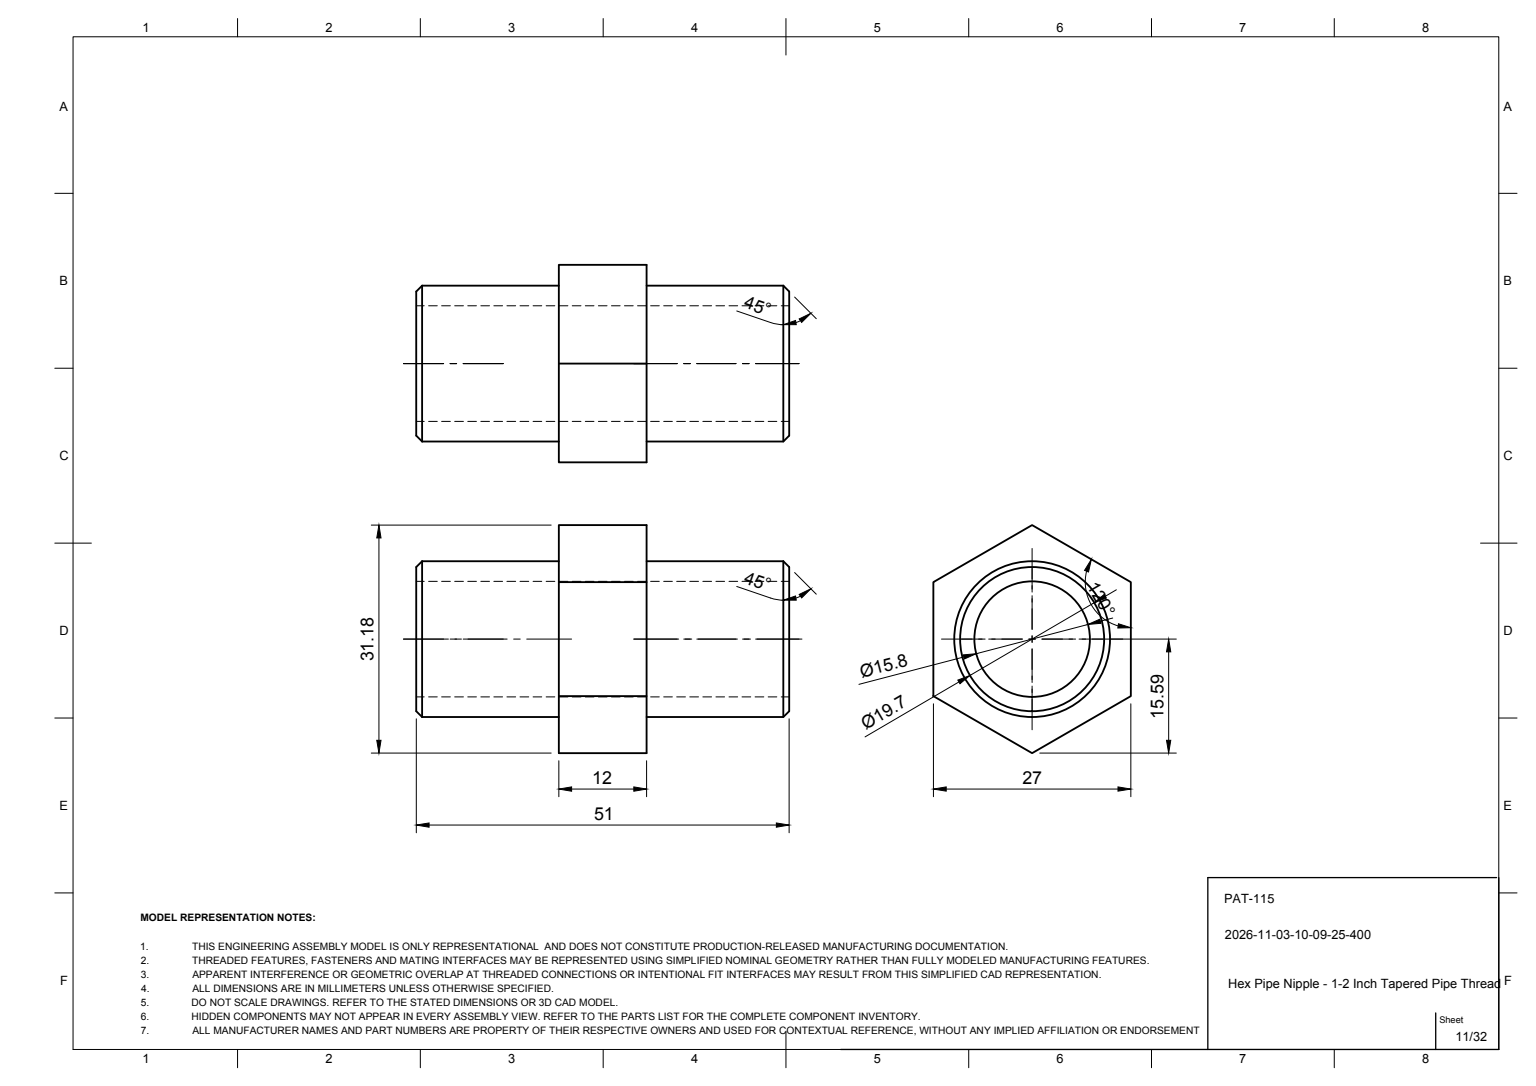
ISO-10303-21;
HEADER;
/* Generated by software containing ST-Developer
 * from STEP Tools, Inc. (www.steptools.com) 
 */

FILE_DESCRIPTION(
/* description */ ('Union bypass pipe loop'),
/* implementation_level */ '2;1');

FILE_NAME(
/* name */ 'Hex Pipe Nipple - 1-2 Inch Tapered Pipe Thread.step',
/* time_stamp */ '2026-10-27T21:00:29-07:00',
/* author */ (''),
/* organization */ (''),
/* preprocessor_version */ 'ST-DEVELOPER v20.2',
/* originating_system */ 'Autodesk Translation Framework v15.17.0.0',
/* authorisation */ '');

FILE_SCHEMA (('AUTOMOTIVE_DESIGN { 1 0 10303 214 3 1 1 }'));
ENDSEC;

DATA;
#10=MECHANICAL_DESIGN_GEOMETRIC_PRESENTATION_REPRESENTATION('',(#465),#10095);
#361=CONICAL_SURFACE('',#6367,1.025,0.785398163397448);
#362=CONICAL_SURFACE('',#6370,1.025,0.785398163397448);
#401=SHAPE_REPRESENTATION_RELATIONSHIP('SRR','None',#10270,#433);
#433=ADVANCED_BREP_SHAPE_REPRESENTATION('',(#495),#10082);
#465=STYLED_ITEM('',(#10486),#495);
#495=MANIFOLD_SOLID_BREP('Body1',#5538);
#595=FACE_BOUND('',#1452,.T.);
#596=FACE_BOUND('',#1454,.T.);
#597=FACE_BOUND('',#1463,.T.);
#598=FACE_BOUND('',#1468,.T.);
#744=PLANE('',#6352);
#745=PLANE('',#6354);
#746=PLANE('',#6356);
#747=PLANE('',#6357);
#748=PLANE('',#6358);
#749=PLANE('',#6359);
#750=PLANE('',#6360);
#751=PLANE('',#6361);
#752=PLANE('',#6364);
#753=PLANE('',#6372);
#1035=FACE_OUTER_BOUND('',#1451,.T.);
#1036=FACE_OUTER_BOUND('',#1453,.T.);
#1037=FACE_OUTER_BOUND('',#1455,.T.);
#1038=FACE_OUTER_BOUND('',#1456,.T.);
#1039=FACE_OUTER_BOUND('',#1457,.T.);
#1040=FACE_OUTER_BOUND('',#1458,.T.);
#1041=FACE_OUTER_BOUND('',#1459,.T.);
#1042=FACE_OUTER_BOUND('',#1460,.T.);
#1043=FACE_OUTER_BOUND('',#1461,.T.);
#1044=FACE_OUTER_BOUND('',#1462,.T.);
#1045=FACE_OUTER_BOUND('',#1464,.T.);
#1046=FACE_OUTER_BOUND('',#1465,.T.);
#1047=FACE_OUTER_BOUND('',#1466,.T.);
#1048=FACE_OUTER_BOUND('',#1467,.T.);
#1049=FACE_OUTER_BOUND('',#1469,.T.);
#1451=EDGE_LOOP('',(#4538,#4539,#4540,#4541,#4542,#4543));
#1452=EDGE_LOOP('',(#4544));
#1453=EDGE_LOOP('',(#4545,#4546,#4547,#4548,#4549,#4550));
#1454=EDGE_LOOP('',(#4551));
#1455=EDGE_LOOP('',(#4552,#4553,#4554,#4555));
#1456=EDGE_LOOP('',(#4556,#4557,#4558,#4559));
#1457=EDGE_LOOP('',(#4560,#4561,#4562,#4563));
#1458=EDGE_LOOP('',(#4564,#4565,#4566,#4567));
#1459=EDGE_LOOP('',(#4568,#4569,#4570,#4571));
#1460=EDGE_LOOP('',(#4572,#4573,#4574,#4575));
#1461=EDGE_LOOP('',(#4576,#4577,#4578,#4579));
#1462=EDGE_LOOP('',(#4580));
#1463=EDGE_LOOP('',(#4581));
#1464=EDGE_LOOP('',(#4582,#4583,#4584,#4585));
#1465=EDGE_LOOP('',(#4586,#4587,#4588,#4589));
#1466=EDGE_LOOP('',(#4590,#4591,#4592,#4593));
#1467=EDGE_LOOP('',(#4594));
#1468=EDGE_LOOP('',(#4595));
#1469=EDGE_LOOP('',(#4596,#4597,#4598,#4599));
#1823=LINE('',#9371,#2199);
#1824=LINE('',#9373,#2200);
#1825=LINE('',#9375,#2201);
#1826=LINE('',#9377,#2202);
#1827=LINE('',#9379,#2203);
#1828=LINE('',#9380,#2204);
#1829=LINE('',#9386,#2205);
#1830=LINE('',#9388,#2206);
#1831=LINE('',#9390,#2207);
#1832=LINE('',#9392,#2208);
#1833=LINE('',#9394,#2209);
#1834=LINE('',#9395,#2210);
#1835=LINE('',#9399,#2211);
#1836=LINE('',#9400,#2212);
#1837=LINE('',#9402,#2213);
#1838=LINE('',#9404,#2214);
#1839=LINE('',#9406,#2215);
#1840=LINE('',#9408,#2216);
#1841=LINE('',#9412,#2217);
#1842=LINE('',#9420,#2218);
#1843=LINE('',#9424,#2219);
#1844=LINE('',#9428,#2220);
#1845=LINE('',#9433,#2221);
#2199=VECTOR('',#7715,1.);
#2200=VECTOR('',#7716,1.);
#2201=VECTOR('',#7717,1.);
#2202=VECTOR('',#7718,1.);
#2203=VECTOR('',#7719,1.);
#2204=VECTOR('',#7720,1.);
#2205=VECTOR('',#7725,1.);
#2206=VECTOR('',#7726,1.);
#2207=VECTOR('',#7727,1.);
#2208=VECTOR('',#7728,1.);
#2209=VECTOR('',#7729,1.);
#2210=VECTOR('',#7730,1.);
#2211=VECTOR('',#7735,1.);
#2212=VECTOR('',#7736,1.);
#2213=VECTOR('',#7739,1.);
#2214=VECTOR('',#7742,1.);
#2215=VECTOR('',#7745,1.);
#2216=VECTOR('',#7748,1.);
#2217=VECTOR('',#7753,1.065);
#2218=VECTOR('',#7764,1.025);
#2219=VECTOR('',#7769,1.065);
#2220=VECTOR('',#7774,1.025);
#2221=VECTOR('',#7781,0.79);
#2547=CIRCLE('',#6353,1.065);
#2548=CIRCLE('',#6355,1.065);
#2549=CIRCLE('',#6363,1.065);
#2550=CIRCLE('',#6365,0.985);
#2551=CIRCLE('',#6366,0.79);
#2552=CIRCLE('',#6369,1.065);
#2553=CIRCLE('',#6371,0.985);
#2554=CIRCLE('',#6373,0.79);
#2892=VERTEX_POINT('',#9369);
#2893=VERTEX_POINT('',#9370);
#2894=VERTEX_POINT('',#9372);
#2895=VERTEX_POINT('',#9374);
#2896=VERTEX_POINT('',#9376);
#2897=VERTEX_POINT('',#9378);
#2898=VERTEX_POINT('',#9381);
#2899=VERTEX_POINT('',#9384);
#2900=VERTEX_POINT('',#9385);
#2901=VERTEX_POINT('',#9387);
#2902=VERTEX_POINT('',#9389);
#2903=VERTEX_POINT('',#9391);
#2904=VERTEX_POINT('',#9393);
#2905=VERTEX_POINT('',#9396);
#2906=VERTEX_POINT('',#9411);
#2907=VERTEX_POINT('',#9415);
#2908=VERTEX_POINT('',#9417);
#2909=VERTEX_POINT('',#9422);
#2910=VERTEX_POINT('',#9426);
#2911=VERTEX_POINT('',#9430);
#3467=EDGE_CURVE('',#2892,#2893,#1823,.T.);
#3468=EDGE_CURVE('',#2893,#2894,#1824,.T.);
#3469=EDGE_CURVE('',#2894,#2895,#1825,.T.);
#3470=EDGE_CURVE('',#2895,#2896,#1826,.T.);
#3471=EDGE_CURVE('',#2896,#2897,#1827,.T.);
#3472=EDGE_CURVE('',#2897,#2892,#1828,.T.);
#3473=EDGE_CURVE('',#2898,#2898,#2547,.T.);
#3474=EDGE_CURVE('',#2899,#2900,#1829,.T.);
#3475=EDGE_CURVE('',#2900,#2901,#1830,.T.);
#3476=EDGE_CURVE('',#2901,#2902,#1831,.T.);
#3477=EDGE_CURVE('',#2902,#2903,#1832,.T.);
#3478=EDGE_CURVE('',#2903,#2904,#1833,.T.);
#3479=EDGE_CURVE('',#2904,#2899,#1834,.T.);
#3480=EDGE_CURVE('',#2905,#2905,#2548,.T.);
#3481=EDGE_CURVE('',#2899,#2893,#1835,.T.);
#3482=EDGE_CURVE('',#2894,#2904,#1836,.T.);
#3483=EDGE_CURVE('',#2895,#2903,#1837,.T.);
#3484=EDGE_CURVE('',#2896,#2902,#1838,.T.);
#3485=EDGE_CURVE('',#2897,#2901,#1839,.T.);
#3486=EDGE_CURVE('',#2892,#2900,#1840,.T.);
#3487=EDGE_CURVE('',#2905,#2906,#1841,.T.);
#3488=EDGE_CURVE('',#2906,#2906,#2549,.T.);
#3489=EDGE_CURVE('',#2907,#2907,#2550,.T.);
#3490=EDGE_CURVE('',#2908,#2908,#2551,.T.);
#3491=EDGE_CURVE('',#2906,#2907,#1842,.T.);
#3492=EDGE_CURVE('',#2909,#2909,#2552,.T.);
#3493=EDGE_CURVE('',#2909,#2898,#1843,.T.);
#3494=EDGE_CURVE('',#2910,#2910,#2553,.T.);
#3495=EDGE_CURVE('',#2910,#2909,#1844,.T.);
#3496=EDGE_CURVE('',#2911,#2911,#2554,.T.);
#3497=EDGE_CURVE('',#2911,#2908,#1845,.T.);
#4538=ORIENTED_EDGE('',*,*,#3467,.T.);
#4539=ORIENTED_EDGE('',*,*,#3468,.T.);
#4540=ORIENTED_EDGE('',*,*,#3469,.T.);
#4541=ORIENTED_EDGE('',*,*,#3470,.T.);
#4542=ORIENTED_EDGE('',*,*,#3471,.T.);
#4543=ORIENTED_EDGE('',*,*,#3472,.T.);
#4544=ORIENTED_EDGE('',*,*,#3473,.F.);
#4545=ORIENTED_EDGE('',*,*,#3474,.T.);
#4546=ORIENTED_EDGE('',*,*,#3475,.T.);
#4547=ORIENTED_EDGE('',*,*,#3476,.T.);
#4548=ORIENTED_EDGE('',*,*,#3477,.T.);
#4549=ORIENTED_EDGE('',*,*,#3478,.T.);
#4550=ORIENTED_EDGE('',*,*,#3479,.T.);
#4551=ORIENTED_EDGE('',*,*,#3480,.F.);
#4552=ORIENTED_EDGE('',*,*,#3481,.F.);
#4553=ORIENTED_EDGE('',*,*,#3479,.F.);
#4554=ORIENTED_EDGE('',*,*,#3482,.F.);
#4555=ORIENTED_EDGE('',*,*,#3468,.F.);
#4556=ORIENTED_EDGE('',*,*,#3482,.T.);
#4557=ORIENTED_EDGE('',*,*,#3478,.F.);
#4558=ORIENTED_EDGE('',*,*,#3483,.F.);
#4559=ORIENTED_EDGE('',*,*,#3469,.F.);
#4560=ORIENTED_EDGE('',*,*,#3483,.T.);
#4561=ORIENTED_EDGE('',*,*,#3477,.F.);
#4562=ORIENTED_EDGE('',*,*,#3484,.F.);
#4563=ORIENTED_EDGE('',*,*,#3470,.F.);
#4564=ORIENTED_EDGE('',*,*,#3484,.T.);
#4565=ORIENTED_EDGE('',*,*,#3476,.F.);
#4566=ORIENTED_EDGE('',*,*,#3485,.F.);
#4567=ORIENTED_EDGE('',*,*,#3471,.F.);
#4568=ORIENTED_EDGE('',*,*,#3485,.T.);
#4569=ORIENTED_EDGE('',*,*,#3475,.F.);
#4570=ORIENTED_EDGE('',*,*,#3486,.F.);
#4571=ORIENTED_EDGE('',*,*,#3472,.F.);
#4572=ORIENTED_EDGE('',*,*,#3486,.T.);
#4573=ORIENTED_EDGE('',*,*,#3474,.F.);
#4574=ORIENTED_EDGE('',*,*,#3481,.T.);
#4575=ORIENTED_EDGE('',*,*,#3467,.F.);
#4576=ORIENTED_EDGE('',*,*,#3480,.T.);
#4577=ORIENTED_EDGE('',*,*,#3487,.T.);
#4578=ORIENTED_EDGE('',*,*,#3488,.T.);
#4579=ORIENTED_EDGE('',*,*,#3487,.F.);
#4580=ORIENTED_EDGE('',*,*,#3489,.F.);
#4581=ORIENTED_EDGE('',*,*,#3490,.T.);
#4582=ORIENTED_EDGE('',*,*,#3488,.F.);
#4583=ORIENTED_EDGE('',*,*,#3491,.T.);
#4584=ORIENTED_EDGE('',*,*,#3489,.T.);
#4585=ORIENTED_EDGE('',*,*,#3491,.F.);
#4586=ORIENTED_EDGE('',*,*,#3492,.F.);
#4587=ORIENTED_EDGE('',*,*,#3493,.T.);
#4588=ORIENTED_EDGE('',*,*,#3473,.T.);
#4589=ORIENTED_EDGE('',*,*,#3493,.F.);
#4590=ORIENTED_EDGE('',*,*,#3494,.F.);
#4591=ORIENTED_EDGE('',*,*,#3495,.T.);
#4592=ORIENTED_EDGE('',*,*,#3492,.T.);
#4593=ORIENTED_EDGE('',*,*,#3495,.F.);
#4594=ORIENTED_EDGE('',*,*,#3494,.T.);
#4595=ORIENTED_EDGE('',*,*,#3496,.F.);
#4596=ORIENTED_EDGE('',*,*,#3496,.T.);
#4597=ORIENTED_EDGE('',*,*,#3497,.T.);
#4598=ORIENTED_EDGE('',*,*,#3490,.F.);
#4599=ORIENTED_EDGE('',*,*,#3497,.F.);
#5155=CYLINDRICAL_SURFACE('',#6362,1.065);
#5156=CYLINDRICAL_SURFACE('',#6368,1.065);
#5157=CYLINDRICAL_SURFACE('',#6374,0.79);
#5384=ADVANCED_FACE('',(#1035,#595),#744,.F.);
#5385=ADVANCED_FACE('',(#1036,#596),#745,.T.);
#5386=ADVANCED_FACE('',(#1037),#746,.T.);
#5387=ADVANCED_FACE('',(#1038),#747,.T.);
#5388=ADVANCED_FACE('',(#1039),#748,.T.);
#5389=ADVANCED_FACE('',(#1040),#749,.T.);
#5390=ADVANCED_FACE('',(#1041),#750,.T.);
#5391=ADVANCED_FACE('',(#1042),#751,.T.);
#5392=ADVANCED_FACE('',(#1043),#5155,.T.);
#5393=ADVANCED_FACE('',(#1044,#597),#752,.T.);
#5394=ADVANCED_FACE('',(#1045),#361,.T.);
#5395=ADVANCED_FACE('',(#1046),#5156,.T.);
#5396=ADVANCED_FACE('',(#1047),#362,.T.);
#5397=ADVANCED_FACE('',(#1048,#598),#753,.T.);
#5398=ADVANCED_FACE('',(#1049),#5157,.F.);
#5538=CLOSED_SHELL('',(#5384,#5385,#5386,#5387,#5388,#5389,#5390,#5391,
#5392,#5393,#5394,#5395,#5396,#5397,#5398));
#6351=AXIS2_PLACEMENT_3D('',#9367,#7711,#7712);
#6352=AXIS2_PLACEMENT_3D('',#9368,#7713,#7714);
#6353=AXIS2_PLACEMENT_3D('',#9382,#7721,#7722);
#6354=AXIS2_PLACEMENT_3D('',#9383,#7723,#7724);
#6355=AXIS2_PLACEMENT_3D('',#9397,#7731,#7732);
#6356=AXIS2_PLACEMENT_3D('',#9398,#7733,#7734);
#6357=AXIS2_PLACEMENT_3D('',#9401,#7737,#7738);
#6358=AXIS2_PLACEMENT_3D('',#9403,#7740,#7741);
#6359=AXIS2_PLACEMENT_3D('',#9405,#7743,#7744);
#6360=AXIS2_PLACEMENT_3D('',#9407,#7746,#7747);
#6361=AXIS2_PLACEMENT_3D('',#9409,#7749,#7750);
#6362=AXIS2_PLACEMENT_3D('',#9410,#7751,#7752);
#6363=AXIS2_PLACEMENT_3D('',#9413,#7754,#7755);
#6364=AXIS2_PLACEMENT_3D('',#9414,#7756,#7757);
#6365=AXIS2_PLACEMENT_3D('',#9416,#7758,#7759);
#6366=AXIS2_PLACEMENT_3D('',#9418,#7760,#7761);
#6367=AXIS2_PLACEMENT_3D('',#9419,#7762,#7763);
#6368=AXIS2_PLACEMENT_3D('',#9421,#7765,#7766);
#6369=AXIS2_PLACEMENT_3D('',#9423,#7767,#7768);
#6370=AXIS2_PLACEMENT_3D('',#9425,#7770,#7771);
#6371=AXIS2_PLACEMENT_3D('',#9427,#7772,#7773);
#6372=AXIS2_PLACEMENT_3D('',#9429,#7775,#7776);
#6373=AXIS2_PLACEMENT_3D('',#9431,#7777,#7778);
#6374=AXIS2_PLACEMENT_3D('',#9432,#7779,#7780);
#7711=DIRECTION('axis',(0.,0.,1.));
#7712=DIRECTION('refdir',(1.,0.,0.));
#7713=DIRECTION('center_axis',(0.,1.,0.));
#7714=DIRECTION('ref_axis',(1.,0.,0.));
#7715=DIRECTION('',(-0.5,0.,0.866025403784439));
#7716=DIRECTION('',(-1.,0.,-2.84883360945713E-16));
#7717=DIRECTION('',(-0.5,0.,-0.866025403784439));
#7718=DIRECTION('',(0.5,0.,-0.866025403784439));
#7719=DIRECTION('',(1.,0.,0.));
#7720=DIRECTION('',(0.5,0.,0.866025403784439));
#7721=DIRECTION('center_axis',(0.,-1.,0.));
#7722=DIRECTION('ref_axis',(1.,0.,0.));
#7723=DIRECTION('center_axis',(0.,1.,0.));
#7724=DIRECTION('ref_axis',(1.,0.,0.));
#7725=DIRECTION('',(0.5,0.,-0.866025403784439));
#7726=DIRECTION('',(-0.5,0.,-0.866025403784439));
#7727=DIRECTION('',(-1.,0.,0.));
#7728=DIRECTION('',(-0.5,0.,0.866025403784439));
#7729=DIRECTION('',(0.5,0.,0.866025403784439));
#7730=DIRECTION('',(1.,0.,2.84883360945713E-16));
#7731=DIRECTION('center_axis',(0.,1.,0.));
#7732=DIRECTION('ref_axis',(1.,0.,0.));
#7733=DIRECTION('center_axis',(-2.84883360945713E-16,0.,1.));
#7734=DIRECTION('ref_axis',(1.,0.,2.84883360945713E-16));
#7735=DIRECTION('',(0.,-1.,0.));
#7736=DIRECTION('',(0.,1.,0.));
#7737=DIRECTION('center_axis',(-0.866025403784439,0.,0.5));
#7738=DIRECTION('ref_axis',(0.5,0.,0.866025403784439));
#7739=DIRECTION('',(0.,1.,0.));
#7740=DIRECTION('center_axis',(-0.866025403784439,0.,-0.5));
#7741=DIRECTION('ref_axis',(-0.5,0.,0.866025403784439));
#7742=DIRECTION('',(0.,1.,0.));
#7743=DIRECTION('center_axis',(0.,0.,-1.));
#7744=DIRECTION('ref_axis',(-1.,0.,0.));
#7745=DIRECTION('',(0.,1.,0.));
#7746=DIRECTION('center_axis',(0.866025403784439,0.,-0.5));
#7747=DIRECTION('ref_axis',(-0.5,0.,-0.866025403784439));
#7748=DIRECTION('',(0.,1.,0.));
#7749=DIRECTION('center_axis',(0.866025403784439,0.,0.5));
#7750=DIRECTION('ref_axis',(0.5,0.,-0.866025403784439));
#7751=DIRECTION('center_axis',(0.,-1.,0.));
#7752=DIRECTION('ref_axis',(1.,0.,0.));
#7753=DIRECTION('',(0.,1.,0.));
#7754=DIRECTION('center_axis',(0.,-1.,0.));
#7755=DIRECTION('ref_axis',(1.,0.,0.));
#7756=DIRECTION('center_axis',(0.,1.,0.));
#7757=DIRECTION('ref_axis',(0.,0.,1.));
#7758=DIRECTION('center_axis',(0.,-1.,0.));
#7759=DIRECTION('ref_axis',(1.,0.,0.));
#7760=DIRECTION('center_axis',(0.,-1.,0.));
#7761=DIRECTION('ref_axis',(1.,0.,0.));
#7762=DIRECTION('center_axis',(0.,-1.,0.));
#7763=DIRECTION('ref_axis',(1.,0.,0.));
#7764=DIRECTION('',(0.707106781186547,0.707106781186548,8.65956056235493E-17));
#7765=DIRECTION('center_axis',(0.,-1.,0.));
#7766=DIRECTION('ref_axis',(1.,0.,0.));
#7767=DIRECTION('center_axis',(0.,-1.,0.));
#7768=DIRECTION('ref_axis',(1.,0.,0.));
#7769=DIRECTION('',(0.,1.,0.));
#7770=DIRECTION('center_axis',(0.,1.,0.));
#7771=DIRECTION('ref_axis',(1.,0.,0.));
#7772=DIRECTION('center_axis',(0.,-1.,0.));
#7773=DIRECTION('ref_axis',(1.,0.,0.));
#7774=DIRECTION('',(-0.707106781186547,0.707106781186548,-8.65956056235493E-17));
#7775=DIRECTION('center_axis',(0.,-1.,0.));
#7776=DIRECTION('ref_axis',(0.,0.,-1.));
#7777=DIRECTION('center_axis',(0.,-1.,0.));
#7778=DIRECTION('ref_axis',(1.,0.,0.));
#7779=DIRECTION('center_axis',(0.,-1.,0.));
#7780=DIRECTION('ref_axis',(1.,0.,0.));
#7781=DIRECTION('',(0.,1.,0.));
#9367=CARTESIAN_POINT('',(0.,0.,0.));
#9368=CARTESIAN_POINT('Origin',(0.,-0.6,0.));
#9369=CARTESIAN_POINT('',(1.55884572681199,-0.6,0.));
#9370=CARTESIAN_POINT('',(0.779422863405995,-0.6,1.35));
#9371=CARTESIAN_POINT('',(0.779422863405995,-0.6,1.35));
#9372=CARTESIAN_POINT('',(-0.779422863405996,-0.6,1.35));
#9373=CARTESIAN_POINT('',(-0.779422863405996,-0.6,1.35));
#9374=CARTESIAN_POINT('',(-1.55884572681199,-0.6,-1.90903542970483E-16));
#9375=CARTESIAN_POINT('',(-1.55884572681199,-0.6,-1.90903542970483E-16));
#9376=CARTESIAN_POINT('',(-0.779422863405995,-0.6,-1.35));
#9377=CARTESIAN_POINT('',(-0.779422863405995,-0.6,-1.35));
#9378=CARTESIAN_POINT('',(0.779422863405995,-0.6,-1.35));
#9379=CARTESIAN_POINT('',(0.779422863405995,-0.6,-1.35));
#9380=CARTESIAN_POINT('',(1.55884572681199,-0.6,0.));
#9381=CARTESIAN_POINT('',(-1.065,-0.6,-1.30424884109193E-16));
#9382=CARTESIAN_POINT('Origin',(0.,-0.6,0.));
#9383=CARTESIAN_POINT('Origin',(0.,0.6,0.));
#9384=CARTESIAN_POINT('',(0.779422863405995,0.6,1.35));
#9385=CARTESIAN_POINT('',(1.55884572681199,0.6,0.));
#9386=CARTESIAN_POINT('',(0.779422863405995,0.6,1.35));
#9387=CARTESIAN_POINT('',(0.779422863405995,0.6,-1.35));
#9388=CARTESIAN_POINT('',(1.55884572681199,0.6,0.));
#9389=CARTESIAN_POINT('',(-0.779422863405995,0.6,-1.35));
#9390=CARTESIAN_POINT('',(0.779422863405995,0.6,-1.35));
#9391=CARTESIAN_POINT('',(-1.55884572681199,0.6,-1.90903542970483E-16));
#9392=CARTESIAN_POINT('',(-0.779422863405995,0.6,-1.35));
#9393=CARTESIAN_POINT('',(-0.779422863405996,0.6,1.35));
#9394=CARTESIAN_POINT('',(-1.55884572681199,0.6,-1.90903542970483E-16));
#9395=CARTESIAN_POINT('',(-0.779422863405996,0.6,1.35));
#9396=CARTESIAN_POINT('',(-1.065,0.6,1.30424884109193E-16));
#9397=CARTESIAN_POINT('Origin',(0.,0.6,0.));
#9398=CARTESIAN_POINT('Origin',(-0.779422863405996,0.,1.35));
#9399=CARTESIAN_POINT('',(0.779422863405995,0.,1.35));
#9400=CARTESIAN_POINT('',(-0.779422863405996,0.,1.35));
#9401=CARTESIAN_POINT('Origin',(-1.55884572681199,0.,-1.90903542970483E-16));
#9402=CARTESIAN_POINT('',(-1.55884572681199,0.,-1.90903542970483E-16));
#9403=CARTESIAN_POINT('Origin',(-0.779422863405995,0.,-1.35));
#9404=CARTESIAN_POINT('',(-0.779422863405995,0.,-1.35));
#9405=CARTESIAN_POINT('Origin',(0.779422863405995,0.,-1.35));
#9406=CARTESIAN_POINT('',(0.779422863405995,0.,-1.35));
#9407=CARTESIAN_POINT('Origin',(1.55884572681199,0.,0.));
#9408=CARTESIAN_POINT('',(1.55884572681199,0.,0.));
#9409=CARTESIAN_POINT('Origin',(0.779422863405995,0.,1.35));
#9410=CARTESIAN_POINT('Origin',(0.,0.,0.));
#9411=CARTESIAN_POINT('',(-1.065,2.47,-1.30424884109193E-16));
#9412=CARTESIAN_POINT('',(-1.065,0.,-1.30424884109193E-16));
#9413=CARTESIAN_POINT('Origin',(0.,2.47,0.));
#9414=CARTESIAN_POINT('Origin',(0.985,2.55,0.));
#9415=CARTESIAN_POINT('',(-0.985,2.55,-1.20627709716014E-16));
#9416=CARTESIAN_POINT('Origin',(0.,2.55,0.));
#9417=CARTESIAN_POINT('',(-0.79,2.55,-9.67470971326409E-17));
#9418=CARTESIAN_POINT('Origin',(0.,2.55,0.));
#9419=CARTESIAN_POINT('Origin',(0.,2.51,0.));
#9420=CARTESIAN_POINT('',(-1.025,2.51,-1.25526296912604E-16));
#9421=CARTESIAN_POINT('Origin',(0.,0.,0.));
#9422=CARTESIAN_POINT('',(-1.065,-2.47,-1.30424884109193E-16));
#9423=CARTESIAN_POINT('Origin',(0.,-2.47,0.));
#9424=CARTESIAN_POINT('',(-1.065,0.,-1.30424884109193E-16));
#9425=CARTESIAN_POINT('Origin',(0.,-2.51,0.));
#9426=CARTESIAN_POINT('',(-0.985,-2.55,-1.20627709716014E-16));
#9427=CARTESIAN_POINT('Origin',(0.,-2.55,0.));
#9428=CARTESIAN_POINT('',(-1.025,-2.51,-1.25526296912604E-16));
#9429=CARTESIAN_POINT('Origin',(0.79,-2.55,0.));
#9430=CARTESIAN_POINT('',(-0.79,-2.55,-9.67470971326409E-17));
#9431=CARTESIAN_POINT('Origin',(0.,-2.55,0.));
#9432=CARTESIAN_POINT('Origin',(0.,0.,0.));
#9433=CARTESIAN_POINT('',(-0.79,0.,-9.67470971326409E-17));
#10045=UNCERTAINTY_MEASURE_WITH_UNIT(LENGTH_MEASURE(0.001),#10096,
'DISTANCE_ACCURACY_VALUE',
'Maximum model space distance between geometric entities at asserted c
onnectivities');
#10058=UNCERTAINTY_MEASURE_WITH_UNIT(LENGTH_MEASURE(0.001),#10096,
'DISTANCE_ACCURACY_VALUE',
'Maximum model space distance between geometric entities at asserted c
onnectivities');
#10082=(
GEOMETRIC_REPRESENTATION_CONTEXT(3)
GLOBAL_UNCERTAINTY_ASSIGNED_CONTEXT((#10045))
GLOBAL_UNIT_ASSIGNED_CONTEXT((#10096,#10098,#10099))
REPRESENTATION_CONTEXT('','3D')
);
#10095=(
GEOMETRIC_REPRESENTATION_CONTEXT(3)
GLOBAL_UNCERTAINTY_ASSIGNED_CONTEXT((#10058))
GLOBAL_UNIT_ASSIGNED_CONTEXT((#10096,#10098,#10099))
REPRESENTATION_CONTEXT('','3D')
);
#10096=(
LENGTH_UNIT()
NAMED_UNIT(*)
SI_UNIT(.CENTI.,.METRE.)
);
#10098=(
NAMED_UNIT(*)
PLANE_ANGLE_UNIT()
SI_UNIT($,.RADIAN.)
);
#10099=(
NAMED_UNIT(*)
SI_UNIT($,.STERADIAN.)
SOLID_ANGLE_UNIT()
);
#10123=SHAPE_DEFINITION_REPRESENTATION(#10194,#10270);
#10194=PRODUCT_DEFINITION_SHAPE('',$,#10307);
#10270=SHAPE_REPRESENTATION('',(#6351),#10082);
#10283=PRODUCT_DEFINITION_CONTEXT('part definition',#10393,'design');
#10307=PRODUCT_DEFINITION(
'Hex Pipe Nipple - 1-2 Inch Tapered Pipe Thread',
'Hex Pipe Nipple - 1-2 Inch Tapered Pipe Thread',#10343,#10283);
#10343=PRODUCT_DEFINITION_FORMATION('',$,#10418);
#10393=APPLICATION_CONTEXT(
'Core Data for Automotive Mechanical Design Process');
#10394=PRODUCT_CONTEXT('part definition',#10393,'mechanical');
#10418=PRODUCT('Hex Pipe Nipple - 1-2 Inch Tapered Pipe Thread',
'Hex Pipe Nipple - 1-2 Inch Tapered Pipe Thread',
'Hex Pipe Nipple - 1-2 Inch Tapered Pipe Thread',(#10394));
#10480=COLOUR_RGB('Light Blue',0.38,0.62,0.78);
#10481=FILL_AREA_STYLE_COLOUR('',#10480);
#10482=FILL_AREA_STYLE('',(#10481));
#10483=SURFACE_STYLE_FILL_AREA(#10482);
#10484=SURFACE_SIDE_STYLE('',(#10483));
#10485=SURFACE_STYLE_USAGE(.BOTH.,#10484);
#10486=PRESENTATION_STYLE_ASSIGNMENT((#10485));
ENDSEC;
END-ISO-10303-21;
